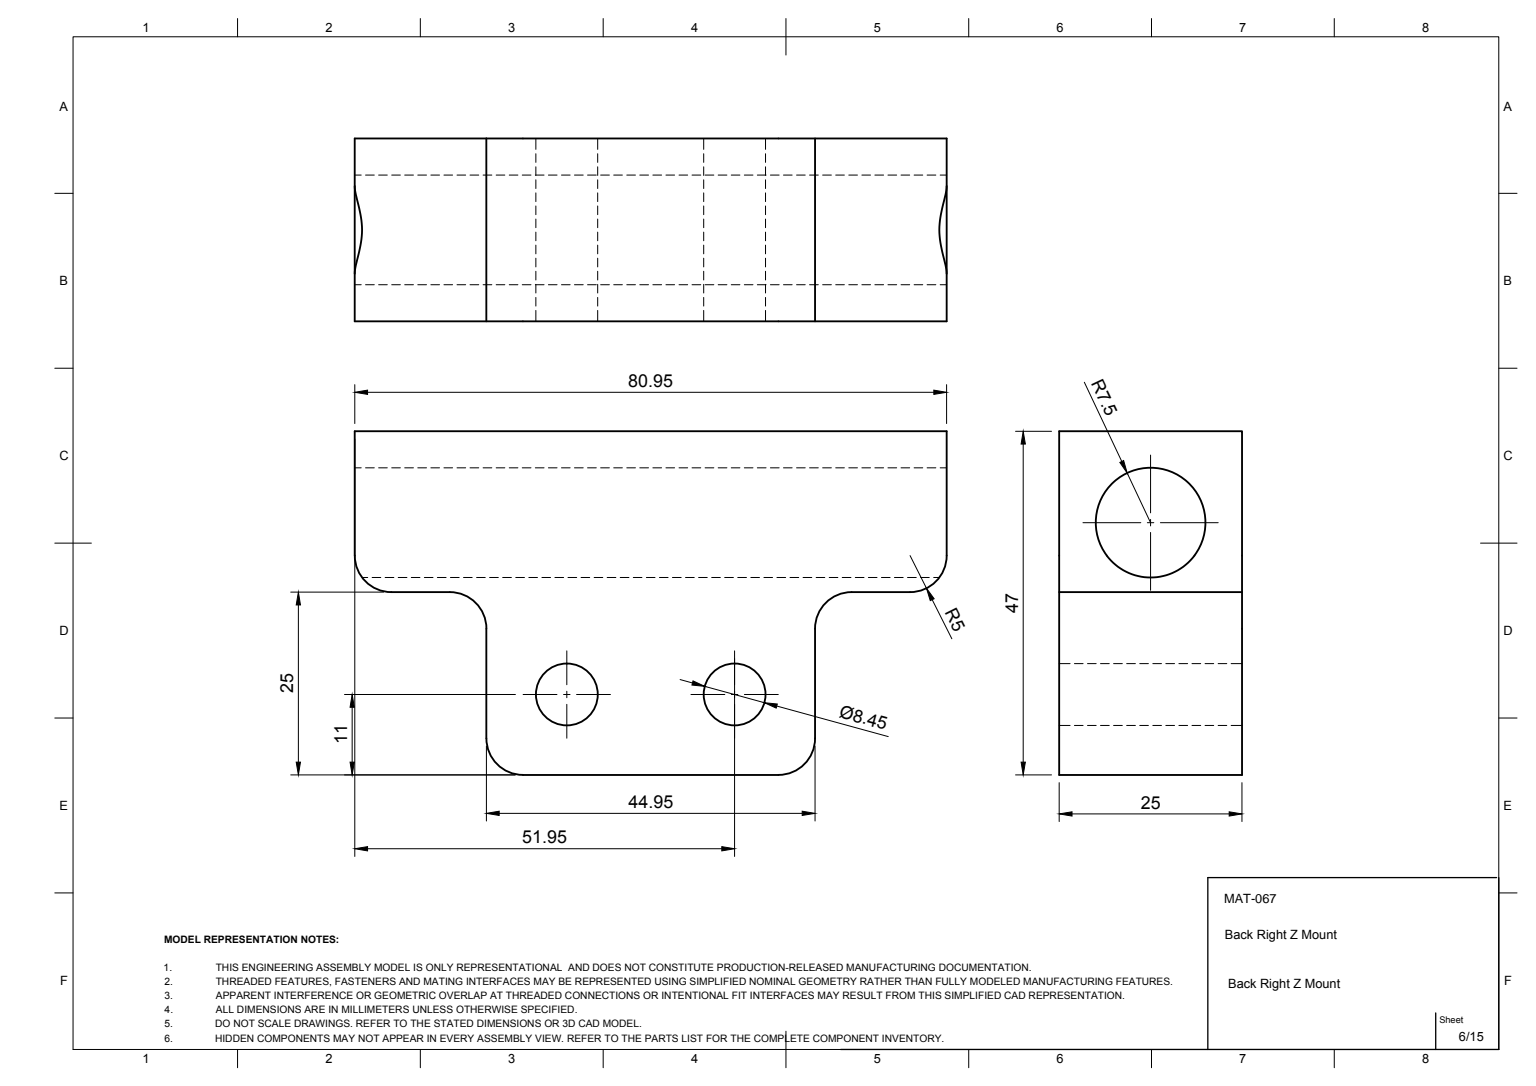
ISO-10303-21;
HEADER;
/* Generated by software containing ST-Developer
 * from STEP Tools, Inc. (www.steptools.com) 
 */

FILE_DESCRIPTION(
/* description */ ('CAx-IF Rec.Pracs.---Representation and Presentation of Product Manufa
cturing Information (PMI)---4.0---2014-10-13'),
/* implementation_level */ '2;1');

FILE_NAME(
/* name */ 'Back Right Z Mount.step',
/* time_stamp */ '2026-10-24T16:02:03-07:00',
/* author */ (''),
/* organization */ (''),
/* preprocessor_version */ 'ST-DEVELOPER v20.2',
/* originating_system */ 'Autodesk Translation Framework v15.17.0.0',
/* authorisation */ '');

FILE_SCHEMA (('AP242_MANAGED_MODEL_BASED_3D_ENGINEERING_MIM_LF { 1 0 10303 442 2 1 4 }'));
ENDSEC;

DATA;
#10=MECHANICAL_DESIGN_GEOMETRIC_PRESENTATION_REPRESENTATION('',(#352),#6348);
#330=SHAPE_REPRESENTATION_RELATIONSHIP('SRR','None',#6480,#341);
#341=ADVANCED_BREP_SHAPE_REPRESENTATION('',(#363),#6328);
#352=STYLED_ITEM('',(#6601),#363);
#363=MANIFOLD_SOLID_BREP('Body1',#3391);
#377=B_SPLINE_CURVE_WITH_KNOTS('',3,(#5673,#5674,#5675,#5676,#5677,#5678,
#5679,#5680,#5681,#5682,#5683,#5684,#5685,#5686,#5687,#5688,#5689,#5690),
 .UNSPECIFIED.,.F.,.F.,(4,2,2,2,2,2,2,2,4),(-2.14352388719531,-2.06484634554612,
-1.76300355616504,-1.61208216147449,-1.46116076678395,-1.31023937209341,
-1.15931797740286,-0.857475188021775,-0.778797646372586),.UNSPECIFIED.);
#378=B_SPLINE_CURVE_WITH_KNOTS('',3,(#5692,#5693,#5694,#5695,#5696,#5697,
#5698,#5699,#5700,#5701,#5702,#5703,#5704,#5705,#5706,#5707,#5708,#5709),
 .UNSPECIFIED.,.F.,.F.,(4,2,2,2,2,2,2,2,4),(-5.06584542076321,-4.98716787911402,
-4.68532508973293,-4.53440369504239,-4.38348230035184,-4.2325609056613,
-4.08163951097076,-3.77979672158967,-3.70111917994048),.UNSPECIFIED.);
#412=CYLINDRICAL_SURFACE('',#3668,0.004225);
#413=CYLINDRICAL_SURFACE('',#3669,0.004225);
#414=CYLINDRICAL_SURFACE('',#3671,0.0075);
#415=CYLINDRICAL_SURFACE('',#3676,0.005);
#416=CYLINDRICAL_SURFACE('',#3677,0.005);
#417=CYLINDRICAL_SURFACE('',#3678,0.005);
#418=CYLINDRICAL_SURFACE('',#3679,0.005);
#419=CYLINDRICAL_SURFACE('',#3680,0.005);
#420=CYLINDRICAL_SURFACE('',#3681,0.005);
#476=FACE_BOUND('',#938,.T.);
#477=FACE_BOUND('',#939,.T.);
#478=FACE_BOUND('',#941,.T.);
#479=FACE_BOUND('',#942,.T.);
#566=CIRCLE('',#3645,0.0075);
#567=CIRCLE('',#3646,0.0075);
#568=CIRCLE('',#3648,0.0075);
#569=CIRCLE('',#3649,0.0075);
#570=CIRCLE('',#3651,0.005);
#571=CIRCLE('',#3652,0.005);
#572=CIRCLE('',#3653,0.005);
#573=CIRCLE('',#3654,0.005);
#574=CIRCLE('',#3655,0.005);
#575=CIRCLE('',#3656,0.005);
#576=CIRCLE('',#3657,0.004225);
#577=CIRCLE('',#3658,0.004225);
#578=CIRCLE('',#3660,0.005);
#579=CIRCLE('',#3661,0.005);
#580=CIRCLE('',#3662,0.005);
#581=CIRCLE('',#3663,0.005);
#582=CIRCLE('',#3664,0.005);
#583=CIRCLE('',#3665,0.005);
#584=CIRCLE('',#3666,0.004225);
#585=CIRCLE('',#3667,0.004225);
#751=FACE_OUTER_BOUND('',#934,.T.);
#752=FACE_OUTER_BOUND('',#935,.T.);
#753=FACE_OUTER_BOUND('',#936,.T.);
#754=FACE_OUTER_BOUND('',#937,.T.);
#755=FACE_OUTER_BOUND('',#940,.T.);
#756=FACE_OUTER_BOUND('',#943,.T.);
#757=FACE_OUTER_BOUND('',#944,.T.);
#758=FACE_OUTER_BOUND('',#945,.T.);
#759=FACE_OUTER_BOUND('',#946,.T.);
#760=FACE_OUTER_BOUND('',#947,.T.);
#761=FACE_OUTER_BOUND('',#948,.T.);
#762=FACE_OUTER_BOUND('',#949,.T.);
#763=FACE_OUTER_BOUND('',#950,.T.);
#764=FACE_OUTER_BOUND('',#951,.T.);
#765=FACE_OUTER_BOUND('',#952,.T.);
#766=FACE_OUTER_BOUND('',#953,.T.);
#767=FACE_OUTER_BOUND('',#954,.T.);
#768=FACE_OUTER_BOUND('',#955,.T.);
#769=FACE_OUTER_BOUND('',#956,.T.);
#934=EDGE_LOOP('',(#2609,#2610,#2611,#2612));
#935=EDGE_LOOP('',(#2613,#2614,#2615,#2616,#2617,#2618,#2619));
#936=EDGE_LOOP('',(#2620,#2621,#2622,#2623,#2624,#2625,#2626));
#937=EDGE_LOOP('',(#2627,#2628,#2629,#2630,#2631,#2632,#2633,#2634,#2635,
#2636,#2637,#2638,#2639,#2640));
#938=EDGE_LOOP('',(#2641));
#939=EDGE_LOOP('',(#2642));
#940=EDGE_LOOP('',(#2643,#2644,#2645,#2646,#2647,#2648,#2649,#2650,#2651,
#2652,#2653,#2654,#2655,#2656));
#941=EDGE_LOOP('',(#2657));
#942=EDGE_LOOP('',(#2658));
#943=EDGE_LOOP('',(#2659,#2660,#2661,#2662));
#944=EDGE_LOOP('',(#2663,#2664,#2665,#2666));
#945=EDGE_LOOP('',(#2667,#2668,#2669,#2670));
#946=EDGE_LOOP('',(#2671,#2672,#2673,#2674,#2675,#2676,#2677,#2678));
#947=EDGE_LOOP('',(#2679,#2680,#2681,#2682));
#948=EDGE_LOOP('',(#2683,#2684,#2685,#2686));
#949=EDGE_LOOP('',(#2687,#2688,#2689,#2690));
#950=EDGE_LOOP('',(#2691,#2692,#2693,#2694));
#951=EDGE_LOOP('',(#2695,#2696,#2697,#2698));
#952=EDGE_LOOP('',(#2699,#2700,#2701,#2702,#2703,#2704));
#953=EDGE_LOOP('',(#2705,#2706,#2707,#2708));
#954=EDGE_LOOP('',(#2709,#2710,#2711,#2712,#2713,#2714));
#955=EDGE_LOOP('',(#2715,#2716,#2717,#2718));
#956=EDGE_LOOP('',(#2719,#2720,#2721,#2722));
#1183=LINE('',#5583,#1416);
#1184=LINE('',#5585,#1417);
#1185=LINE('',#5587,#1418);
#1186=LINE('',#5588,#1419);
#1187=LINE('',#5592,#1420);
#1188=LINE('',#5594,#1421);
#1189=LINE('',#5600,#1422);
#1190=LINE('',#5602,#1423);
#1191=LINE('',#5603,#1424);
#1192=LINE('',#5607,#1425);
#1193=LINE('',#5609,#1426);
#1194=LINE('',#5615,#1427);
#1195=LINE('',#5617,#1428);
#1196=LINE('',#5618,#1429);
#1197=LINE('',#5623,#1430);
#1198=LINE('',#5627,#1431);
#1199=LINE('',#5629,#1432);
#1200=LINE('',#5633,#1433);
#1201=LINE('',#5637,#1434);
#1202=LINE('',#5646,#1435);
#1203=LINE('',#5651,#1436);
#1204=LINE('',#5655,#1437);
#1205=LINE('',#5657,#1438);
#1206=LINE('',#5661,#1439);
#1207=LINE('',#5668,#1440);
#1208=LINE('',#5670,#1441);
#1209=LINE('',#5691,#1442);
#1210=LINE('',#5711,#1443);
#1211=LINE('',#5712,#1444);
#1212=LINE('',#5714,#1445);
#1213=LINE('',#5715,#1446);
#1214=LINE('',#5717,#1447);
#1215=LINE('',#5718,#1448);
#1216=LINE('',#5720,#1449);
#1217=LINE('',#5721,#1450);
#1416=VECTOR('',#4331,1.);
#1417=VECTOR('',#4332,1.);
#1418=VECTOR('',#4333,1.);
#1419=VECTOR('',#4334,1.);
#1420=VECTOR('',#4337,1.);
#1421=VECTOR('',#4338,1.);
#1422=VECTOR('',#4343,1.);
#1423=VECTOR('',#4344,1.);
#1424=VECTOR('',#4345,1.);
#1425=VECTOR('',#4348,1.);
#1426=VECTOR('',#4349,1.);
#1427=VECTOR('',#4354,1.);
#1428=VECTOR('',#4355,1.);
#1429=VECTOR('',#4356,1.);
#1430=VECTOR('',#4361,1.);
#1431=VECTOR('',#4364,1.);
#1432=VECTOR('',#4367,1.);
#1433=VECTOR('',#4370,1.);
#1434=VECTOR('',#4373,1.);
#1435=VECTOR('',#4382,1.);
#1436=VECTOR('',#4387,1.);
#1437=VECTOR('',#4390,1.);
#1438=VECTOR('',#4393,1.);
#1439=VECTOR('',#4396,1.);
#1440=VECTOR('',#4405,0.004225);
#1441=VECTOR('',#4408,0.004225);
#1442=VECTOR('',#4413,0.0075);
#1443=VECTOR('',#4416,1.);
#1444=VECTOR('',#4417,1.);
#1445=VECTOR('',#4420,1.);
#1446=VECTOR('',#4421,1.);
#1447=VECTOR('',#4424,1.);
#1448=VECTOR('',#4425,1.);
#1449=VECTOR('',#4428,1.);
#1450=VECTOR('',#4429,1.);
#1658=VERTEX_POINT('',#5581);
#1659=VERTEX_POINT('',#5582);
#1660=VERTEX_POINT('',#5584);
#1661=VERTEX_POINT('',#5586);
#1662=VERTEX_POINT('',#5590);
#1663=VERTEX_POINT('',#5591);
#1664=VERTEX_POINT('',#5593);
#1665=VERTEX_POINT('',#5595);
#1666=VERTEX_POINT('',#5597);
#1667=VERTEX_POINT('',#5599);
#1668=VERTEX_POINT('',#5601);
#1669=VERTEX_POINT('',#5605);
#1670=VERTEX_POINT('',#5606);
#1671=VERTEX_POINT('',#5608);
#1672=VERTEX_POINT('',#5610);
#1673=VERTEX_POINT('',#5612);
#1674=VERTEX_POINT('',#5614);
#1675=VERTEX_POINT('',#5616);
#1676=VERTEX_POINT('',#5620);
#1677=VERTEX_POINT('',#5622);
#1678=VERTEX_POINT('',#5624);
#1679=VERTEX_POINT('',#5626);
#1680=VERTEX_POINT('',#5630);
#1681=VERTEX_POINT('',#5632);
#1682=VERTEX_POINT('',#5634);
#1683=VERTEX_POINT('',#5636);
#1684=VERTEX_POINT('',#5639);
#1685=VERTEX_POINT('',#5641);
#1686=VERTEX_POINT('',#5644);
#1687=VERTEX_POINT('',#5645);
#1688=VERTEX_POINT('',#5648);
#1689=VERTEX_POINT('',#5650);
#1690=VERTEX_POINT('',#5652);
#1691=VERTEX_POINT('',#5654);
#1692=VERTEX_POINT('',#5658);
#1693=VERTEX_POINT('',#5660);
#1694=VERTEX_POINT('',#5663);
#1695=VERTEX_POINT('',#5665);
#2003=EDGE_CURVE('',#1658,#1659,#1183,.T.);
#2004=EDGE_CURVE('',#1659,#1660,#1184,.T.);
#2005=EDGE_CURVE('',#1661,#1660,#1185,.T.);
#2006=EDGE_CURVE('',#1661,#1658,#1186,.F.);
#2007=EDGE_CURVE('',#1662,#1663,#1187,.T.);
#2008=EDGE_CURVE('',#1662,#1664,#1188,.F.);
#2009=EDGE_CURVE('',#1664,#1665,#566,.T.);
#2010=EDGE_CURVE('',#1665,#1666,#567,.T.);
#2011=EDGE_CURVE('',#1666,#1667,#1189,.F.);
#2012=EDGE_CURVE('',#1667,#1668,#1190,.T.);
#2013=EDGE_CURVE('',#1663,#1668,#1191,.T.);
#2014=EDGE_CURVE('',#1669,#1670,#1192,.T.);
#2015=EDGE_CURVE('',#1669,#1671,#1193,.T.);
#2016=EDGE_CURVE('',#1672,#1671,#568,.T.);
#2017=EDGE_CURVE('',#1673,#1672,#569,.T.);
#2018=EDGE_CURVE('',#1673,#1674,#1194,.T.);
#2019=EDGE_CURVE('',#1674,#1675,#1195,.T.);
#2020=EDGE_CURVE('',#1675,#1670,#1196,.T.);
#2021=EDGE_CURVE('',#1660,#1676,#570,.T.);
#2022=EDGE_CURVE('',#1676,#1677,#1197,.T.);
#2023=EDGE_CURVE('',#1677,#1678,#571,.F.);
#2024=EDGE_CURVE('',#1679,#1678,#1198,.T.);
#2025=EDGE_CURVE('',#1679,#1662,#572,.T.);
#2026=EDGE_CURVE('',#1675,#1663,#1199,.T.);
#2027=EDGE_CURVE('',#1674,#1680,#573,.T.);
#2028=EDGE_CURVE('',#1680,#1681,#1200,.T.);
#2029=EDGE_CURVE('',#1681,#1682,#574,.F.);
#2030=EDGE_CURVE('',#1683,#1682,#1201,.T.);
#2031=EDGE_CURVE('',#1683,#1661,#575,.T.);
#2032=EDGE_CURVE('',#1684,#1684,#576,.T.);
#2033=EDGE_CURVE('',#1685,#1685,#577,.T.);
#2034=EDGE_CURVE('',#1686,#1687,#1202,.T.);
#2035=EDGE_CURVE('',#1686,#1659,#578,.F.);
#2036=EDGE_CURVE('',#1658,#1688,#579,.F.);
#2037=EDGE_CURVE('',#1688,#1689,#1203,.T.);
#2038=EDGE_CURVE('',#1689,#1690,#580,.T.);
#2039=EDGE_CURVE('',#1691,#1690,#1204,.T.);
#2040=EDGE_CURVE('',#1691,#1669,#581,.F.);
#2041=EDGE_CURVE('',#1670,#1668,#1205,.T.);
#2042=EDGE_CURVE('',#1667,#1692,#582,.F.);
#2043=EDGE_CURVE('',#1692,#1693,#1206,.T.);
#2044=EDGE_CURVE('',#1693,#1687,#583,.T.);
#2045=EDGE_CURVE('',#1694,#1694,#584,.T.);
#2046=EDGE_CURVE('',#1695,#1695,#585,.T.);
#2047=EDGE_CURVE('',#1684,#1694,#1207,.T.);
#2048=EDGE_CURVE('',#1685,#1695,#1208,.T.);
#2049=EDGE_CURVE('',#1664,#1666,#377,.T.);
#2050=EDGE_CURVE('',#1665,#1672,#1209,.T.);
#2051=EDGE_CURVE('',#1671,#1673,#378,.T.);
#2052=EDGE_CURVE('',#1676,#1686,#1210,.F.);
#2053=EDGE_CURVE('',#1687,#1677,#1211,.T.);
#2054=EDGE_CURVE('',#1692,#1679,#1212,.T.);
#2055=EDGE_CURVE('',#1678,#1693,#1213,.F.);
#2056=EDGE_CURVE('',#1682,#1689,#1214,.F.);
#2057=EDGE_CURVE('',#1688,#1683,#1215,.T.);
#2058=EDGE_CURVE('',#1680,#1691,#1216,.F.);
#2059=EDGE_CURVE('',#1690,#1681,#1217,.T.);
#2609=ORIENTED_EDGE('',*,*,#2003,.T.);
#2610=ORIENTED_EDGE('',*,*,#2004,.T.);
#2611=ORIENTED_EDGE('',*,*,#2005,.F.);
#2612=ORIENTED_EDGE('',*,*,#2006,.T.);
#2613=ORIENTED_EDGE('',*,*,#2007,.F.);
#2614=ORIENTED_EDGE('',*,*,#2008,.T.);
#2615=ORIENTED_EDGE('',*,*,#2009,.T.);
#2616=ORIENTED_EDGE('',*,*,#2010,.T.);
#2617=ORIENTED_EDGE('',*,*,#2011,.T.);
#2618=ORIENTED_EDGE('',*,*,#2012,.T.);
#2619=ORIENTED_EDGE('',*,*,#2013,.F.);
#2620=ORIENTED_EDGE('',*,*,#2014,.F.);
#2621=ORIENTED_EDGE('',*,*,#2015,.T.);
#2622=ORIENTED_EDGE('',*,*,#2016,.F.);
#2623=ORIENTED_EDGE('',*,*,#2017,.F.);
#2624=ORIENTED_EDGE('',*,*,#2018,.T.);
#2625=ORIENTED_EDGE('',*,*,#2019,.T.);
#2626=ORIENTED_EDGE('',*,*,#2020,.T.);
#2627=ORIENTED_EDGE('',*,*,#2005,.T.);
#2628=ORIENTED_EDGE('',*,*,#2021,.T.);
#2629=ORIENTED_EDGE('',*,*,#2022,.T.);
#2630=ORIENTED_EDGE('',*,*,#2023,.T.);
#2631=ORIENTED_EDGE('',*,*,#2024,.F.);
#2632=ORIENTED_EDGE('',*,*,#2025,.T.);
#2633=ORIENTED_EDGE('',*,*,#2007,.T.);
#2634=ORIENTED_EDGE('',*,*,#2026,.F.);
#2635=ORIENTED_EDGE('',*,*,#2019,.F.);
#2636=ORIENTED_EDGE('',*,*,#2027,.T.);
#2637=ORIENTED_EDGE('',*,*,#2028,.T.);
#2638=ORIENTED_EDGE('',*,*,#2029,.T.);
#2639=ORIENTED_EDGE('',*,*,#2030,.F.);
#2640=ORIENTED_EDGE('',*,*,#2031,.T.);
#2641=ORIENTED_EDGE('',*,*,#2032,.F.);
#2642=ORIENTED_EDGE('',*,*,#2033,.F.);
#2643=ORIENTED_EDGE('',*,*,#2034,.F.);
#2644=ORIENTED_EDGE('',*,*,#2035,.T.);
#2645=ORIENTED_EDGE('',*,*,#2003,.F.);
#2646=ORIENTED_EDGE('',*,*,#2036,.T.);
#2647=ORIENTED_EDGE('',*,*,#2037,.T.);
#2648=ORIENTED_EDGE('',*,*,#2038,.T.);
#2649=ORIENTED_EDGE('',*,*,#2039,.F.);
#2650=ORIENTED_EDGE('',*,*,#2040,.T.);
#2651=ORIENTED_EDGE('',*,*,#2014,.T.);
#2652=ORIENTED_EDGE('',*,*,#2041,.T.);
#2653=ORIENTED_EDGE('',*,*,#2012,.F.);
#2654=ORIENTED_EDGE('',*,*,#2042,.T.);
#2655=ORIENTED_EDGE('',*,*,#2043,.T.);
#2656=ORIENTED_EDGE('',*,*,#2044,.T.);
#2657=ORIENTED_EDGE('',*,*,#2045,.T.);
#2658=ORIENTED_EDGE('',*,*,#2046,.T.);
#2659=ORIENTED_EDGE('',*,*,#2032,.T.);
#2660=ORIENTED_EDGE('',*,*,#2047,.T.);
#2661=ORIENTED_EDGE('',*,*,#2045,.F.);
#2662=ORIENTED_EDGE('',*,*,#2047,.F.);
#2663=ORIENTED_EDGE('',*,*,#2033,.T.);
#2664=ORIENTED_EDGE('',*,*,#2048,.T.);
#2665=ORIENTED_EDGE('',*,*,#2046,.F.);
#2666=ORIENTED_EDGE('',*,*,#2048,.F.);
#2667=ORIENTED_EDGE('',*,*,#2041,.F.);
#2668=ORIENTED_EDGE('',*,*,#2020,.F.);
#2669=ORIENTED_EDGE('',*,*,#2026,.T.);
#2670=ORIENTED_EDGE('',*,*,#2013,.T.);
#2671=ORIENTED_EDGE('',*,*,#2009,.F.);
#2672=ORIENTED_EDGE('',*,*,#2049,.T.);
#2673=ORIENTED_EDGE('',*,*,#2010,.F.);
#2674=ORIENTED_EDGE('',*,*,#2050,.T.);
#2675=ORIENTED_EDGE('',*,*,#2016,.T.);
#2676=ORIENTED_EDGE('',*,*,#2051,.T.);
#2677=ORIENTED_EDGE('',*,*,#2017,.T.);
#2678=ORIENTED_EDGE('',*,*,#2050,.F.);
#2679=ORIENTED_EDGE('',*,*,#2022,.F.);
#2680=ORIENTED_EDGE('',*,*,#2052,.T.);
#2681=ORIENTED_EDGE('',*,*,#2034,.T.);
#2682=ORIENTED_EDGE('',*,*,#2053,.T.);
#2683=ORIENTED_EDGE('',*,*,#2043,.F.);
#2684=ORIENTED_EDGE('',*,*,#2054,.T.);
#2685=ORIENTED_EDGE('',*,*,#2024,.T.);
#2686=ORIENTED_EDGE('',*,*,#2055,.T.);
#2687=ORIENTED_EDGE('',*,*,#2030,.T.);
#2688=ORIENTED_EDGE('',*,*,#2056,.T.);
#2689=ORIENTED_EDGE('',*,*,#2037,.F.);
#2690=ORIENTED_EDGE('',*,*,#2057,.T.);
#2691=ORIENTED_EDGE('',*,*,#2028,.F.);
#2692=ORIENTED_EDGE('',*,*,#2058,.T.);
#2693=ORIENTED_EDGE('',*,*,#2039,.T.);
#2694=ORIENTED_EDGE('',*,*,#2059,.T.);
#2695=ORIENTED_EDGE('',*,*,#2035,.F.);
#2696=ORIENTED_EDGE('',*,*,#2052,.F.);
#2697=ORIENTED_EDGE('',*,*,#2021,.F.);
#2698=ORIENTED_EDGE('',*,*,#2004,.F.);
#2699=ORIENTED_EDGE('',*,*,#2049,.F.);
#2700=ORIENTED_EDGE('',*,*,#2008,.F.);
#2701=ORIENTED_EDGE('',*,*,#2025,.F.);
#2702=ORIENTED_EDGE('',*,*,#2054,.F.);
#2703=ORIENTED_EDGE('',*,*,#2042,.F.);
#2704=ORIENTED_EDGE('',*,*,#2011,.F.);
#2705=ORIENTED_EDGE('',*,*,#2044,.F.);
#2706=ORIENTED_EDGE('',*,*,#2055,.F.);
#2707=ORIENTED_EDGE('',*,*,#2023,.F.);
#2708=ORIENTED_EDGE('',*,*,#2053,.F.);
#2709=ORIENTED_EDGE('',*,*,#2040,.F.);
#2710=ORIENTED_EDGE('',*,*,#2058,.F.);
#2711=ORIENTED_EDGE('',*,*,#2027,.F.);
#2712=ORIENTED_EDGE('',*,*,#2018,.F.);
#2713=ORIENTED_EDGE('',*,*,#2051,.F.);
#2714=ORIENTED_EDGE('',*,*,#2015,.F.);
#2715=ORIENTED_EDGE('',*,*,#2038,.F.);
#2716=ORIENTED_EDGE('',*,*,#2056,.F.);
#2717=ORIENTED_EDGE('',*,*,#2029,.F.);
#2718=ORIENTED_EDGE('',*,*,#2059,.F.);
#2719=ORIENTED_EDGE('',*,*,#2036,.F.);
#2720=ORIENTED_EDGE('',*,*,#2006,.F.);
#2721=ORIENTED_EDGE('',*,*,#2031,.F.);
#2722=ORIENTED_EDGE('',*,*,#2057,.F.);
#3167=PLANE('',#3643);
#3168=PLANE('',#3644);
#3169=PLANE('',#3647);
#3170=PLANE('',#3650);
#3171=PLANE('',#3659);
#3172=PLANE('',#3670);
#3173=PLANE('',#3672);
#3174=PLANE('',#3673);
#3175=PLANE('',#3674);
#3176=PLANE('',#3675);
#3274=ADVANCED_FACE('',(#751),#3167,.F.);
#3275=ADVANCED_FACE('',(#752),#3168,.F.);
#3276=ADVANCED_FACE('',(#753),#3169,.T.);
#3277=ADVANCED_FACE('',(#754,#476,#477),#3170,.T.);
#3278=ADVANCED_FACE('',(#755,#478,#479),#3171,.F.);
#3279=ADVANCED_FACE('',(#756),#412,.F.);
#3280=ADVANCED_FACE('',(#757),#413,.F.);
#3281=ADVANCED_FACE('',(#758),#3172,.T.);
#3282=ADVANCED_FACE('',(#759),#414,.F.);
#3283=ADVANCED_FACE('',(#760),#3173,.T.);
#3284=ADVANCED_FACE('',(#761),#3174,.F.);
#3285=ADVANCED_FACE('',(#762),#3175,.F.);
#3286=ADVANCED_FACE('',(#763),#3176,.T.);
#3287=ADVANCED_FACE('',(#764),#415,.T.);
#3288=ADVANCED_FACE('',(#765),#416,.T.);
#3289=ADVANCED_FACE('',(#766),#417,.F.);
#3290=ADVANCED_FACE('',(#767),#418,.T.);
#3291=ADVANCED_FACE('',(#768),#419,.F.);
#3292=ADVANCED_FACE('',(#769),#420,.T.);
#3391=CLOSED_SHELL('',(#3274,#3275,#3276,#3277,#3278,#3279,#3280,#3281,
#3282,#3283,#3284,#3285,#3286,#3287,#3288,#3289,#3290,#3291,#3292));
#3642=AXIS2_PLACEMENT_3D('',#5579,#4327,#4328);
#3643=AXIS2_PLACEMENT_3D('',#5580,#4329,#4330);
#3644=AXIS2_PLACEMENT_3D('',#5589,#4335,#4336);
#3645=AXIS2_PLACEMENT_3D('',#5596,#4339,#4340);
#3646=AXIS2_PLACEMENT_3D('',#5598,#4341,#4342);
#3647=AXIS2_PLACEMENT_3D('',#5604,#4346,#4347);
#3648=AXIS2_PLACEMENT_3D('',#5611,#4350,#4351);
#3649=AXIS2_PLACEMENT_3D('',#5613,#4352,#4353);
#3650=AXIS2_PLACEMENT_3D('',#5619,#4357,#4358);
#3651=AXIS2_PLACEMENT_3D('',#5621,#4359,#4360);
#3652=AXIS2_PLACEMENT_3D('',#5625,#4362,#4363);
#3653=AXIS2_PLACEMENT_3D('',#5628,#4365,#4366);
#3654=AXIS2_PLACEMENT_3D('',#5631,#4368,#4369);
#3655=AXIS2_PLACEMENT_3D('',#5635,#4371,#4372);
#3656=AXIS2_PLACEMENT_3D('',#5638,#4374,#4375);
#3657=AXIS2_PLACEMENT_3D('',#5640,#4376,#4377);
#3658=AXIS2_PLACEMENT_3D('',#5642,#4378,#4379);
#3659=AXIS2_PLACEMENT_3D('',#5643,#4380,#4381);
#3660=AXIS2_PLACEMENT_3D('',#5647,#4383,#4384);
#3661=AXIS2_PLACEMENT_3D('',#5649,#4385,#4386);
#3662=AXIS2_PLACEMENT_3D('',#5653,#4388,#4389);
#3663=AXIS2_PLACEMENT_3D('',#5656,#4391,#4392);
#3664=AXIS2_PLACEMENT_3D('',#5659,#4394,#4395);
#3665=AXIS2_PLACEMENT_3D('',#5662,#4397,#4398);
#3666=AXIS2_PLACEMENT_3D('',#5664,#4399,#4400);
#3667=AXIS2_PLACEMENT_3D('',#5666,#4401,#4402);
#3668=AXIS2_PLACEMENT_3D('',#5667,#4403,#4404);
#3669=AXIS2_PLACEMENT_3D('',#5669,#4406,#4407);
#3670=AXIS2_PLACEMENT_3D('',#5671,#4409,#4410);
#3671=AXIS2_PLACEMENT_3D('',#5672,#4411,#4412);
#3672=AXIS2_PLACEMENT_3D('',#5710,#4414,#4415);
#3673=AXIS2_PLACEMENT_3D('',#5713,#4418,#4419);
#3674=AXIS2_PLACEMENT_3D('',#5716,#4422,#4423);
#3675=AXIS2_PLACEMENT_3D('',#5719,#4426,#4427);
#3676=AXIS2_PLACEMENT_3D('',#5722,#4430,#4431);
#3677=AXIS2_PLACEMENT_3D('',#5723,#4432,#4433);
#3678=AXIS2_PLACEMENT_3D('',#5724,#4434,#4435);
#3679=AXIS2_PLACEMENT_3D('',#5725,#4436,#4437);
#3680=AXIS2_PLACEMENT_3D('',#5726,#4438,#4439);
#3681=AXIS2_PLACEMENT_3D('',#5727,#4440,#4441);
#4327=DIRECTION('axis',(0.,0.,1.));
#4328=DIRECTION('refdir',(1.,0.,0.));
#4329=DIRECTION('center_axis',(-1.,0.,0.));
#4330=DIRECTION('ref_axis',(0.,0.,-1.));
#4331=DIRECTION('',(0.,8.57182693503055E-17,-1.));
#4332=DIRECTION('',(0.,1.,8.57182693503055E-17));
#4333=DIRECTION('',(0.,8.57182693503055E-17,-1.));
#4334=DIRECTION('',(0.,1.,8.57182693503055E-17));
#4335=DIRECTION('center_axis',(0.,-8.57182693503055E-17,1.));
#4336=DIRECTION('ref_axis',(0.,1.,8.57182693503055E-17));
#4337=DIRECTION('',(-1.,0.,0.));
#4338=DIRECTION('',(0.,1.,8.57182693503055E-17));
#4339=DIRECTION('center_axis',(0.,-8.57182693503055E-17,1.));
#4340=DIRECTION('ref_axis',(0.,1.,8.57182693503055E-17));
#4341=DIRECTION('center_axis',(0.,-8.57182693503055E-17,1.));
#4342=DIRECTION('ref_axis',(0.,1.,8.57182693503055E-17));
#4343=DIRECTION('',(0.,1.,8.57182693503055E-17));
#4344=DIRECTION('',(-1.,0.,0.));
#4345=DIRECTION('',(0.,-1.,-8.57182693503055E-17));
#4346=DIRECTION('center_axis',(0.,-8.57182693503055E-17,1.));
#4347=DIRECTION('ref_axis',(0.,1.,8.57182693503055E-17));
#4348=DIRECTION('',(-1.,0.,0.));
#4349=DIRECTION('',(0.,1.,8.57182693503055E-17));
#4350=DIRECTION('center_axis',(0.,-8.57182693503055E-17,1.));
#4351=DIRECTION('ref_axis',(0.,1.,8.57182693503055E-17));
#4352=DIRECTION('center_axis',(0.,-8.57182693503055E-17,1.));
#4353=DIRECTION('ref_axis',(0.,1.,8.57182693503055E-17));
#4354=DIRECTION('',(0.,1.,8.57182693503055E-17));
#4355=DIRECTION('',(-1.,0.,0.));
#4356=DIRECTION('',(0.,-1.,-8.57182693503055E-17));
#4357=DIRECTION('center_axis',(0.,1.,8.57182693503055E-17));
#4358=DIRECTION('ref_axis',(-1.,0.,0.));
#4359=DIRECTION('center_axis',(0.,1.,8.57182693503055E-17));
#4360=DIRECTION('ref_axis',(0.,8.57182693503055E-17,-1.));
#4361=DIRECTION('',(-1.,0.,0.));
#4362=DIRECTION('center_axis',(0.,1.,8.57182693503055E-17));
#4363=DIRECTION('ref_axis',(0.,8.57182693503055E-17,-1.));
#4364=DIRECTION('',(0.,-8.57182693503055E-17,1.));
#4365=DIRECTION('center_axis',(0.,1.,8.57182693503055E-17));
#4366=DIRECTION('ref_axis',(0.,8.57182693503055E-17,-1.));
#4367=DIRECTION('',(0.,8.57182693503055E-17,-1.));
#4368=DIRECTION('center_axis',(0.,1.,8.57182693503055E-17));
#4369=DIRECTION('ref_axis',(0.,8.57182693503055E-17,-1.));
#4370=DIRECTION('',(0.,8.57182693503055E-17,-1.));
#4371=DIRECTION('center_axis',(0.,1.,8.57182693503055E-17));
#4372=DIRECTION('ref_axis',(0.,8.57182693503055E-17,-1.));
#4373=DIRECTION('',(-1.,0.,0.));
#4374=DIRECTION('center_axis',(0.,1.,8.57182693503055E-17));
#4375=DIRECTION('ref_axis',(0.,8.57182693503055E-17,-1.));
#4376=DIRECTION('center_axis',(0.,1.,8.57182693503055E-17));
#4377=DIRECTION('ref_axis',(0.,8.57182693503055E-17,-1.));
#4378=DIRECTION('center_axis',(0.,1.,8.57182693503055E-17));
#4379=DIRECTION('ref_axis',(0.,8.57182693503055E-17,-1.));
#4380=DIRECTION('center_axis',(0.,1.,8.57182693503055E-17));
#4381=DIRECTION('ref_axis',(-1.,0.,0.));
#4382=DIRECTION('',(-1.,0.,0.));
#4383=DIRECTION('center_axis',(0.,1.,8.57182693503055E-17));
#4384=DIRECTION('ref_axis',(0.,8.57182693503055E-17,-1.));
#4385=DIRECTION('center_axis',(0.,1.,8.57182693503055E-17));
#4386=DIRECTION('ref_axis',(0.,8.57182693503055E-17,-1.));
#4387=DIRECTION('',(-1.,0.,0.));
#4388=DIRECTION('center_axis',(0.,1.,8.57182693503055E-17));
#4389=DIRECTION('ref_axis',(0.,8.57182693503055E-17,-1.));
#4390=DIRECTION('',(0.,8.57182693503055E-17,-1.));
#4391=DIRECTION('center_axis',(0.,1.,8.57182693503055E-17));
#4392=DIRECTION('ref_axis',(0.,8.57182693503055E-17,-1.));
#4393=DIRECTION('',(0.,8.57182693503055E-17,-1.));
#4394=DIRECTION('center_axis',(0.,1.,8.57182693503055E-17));
#4395=DIRECTION('ref_axis',(0.,8.57182693503055E-17,-1.));
#4396=DIRECTION('',(0.,-8.57182693503055E-17,1.));
#4397=DIRECTION('center_axis',(0.,1.,8.57182693503055E-17));
#4398=DIRECTION('ref_axis',(0.,8.57182693503055E-17,-1.));
#4399=DIRECTION('center_axis',(0.,1.,8.57182693503055E-17));
#4400=DIRECTION('ref_axis',(0.,8.57182693503055E-17,-1.));
#4401=DIRECTION('center_axis',(0.,1.,8.57182693503055E-17));
#4402=DIRECTION('ref_axis',(0.,8.57182693503055E-17,-1.));
#4403=DIRECTION('center_axis',(0.,-1.,-8.57182693503055E-17));
#4404=DIRECTION('ref_axis',(0.,-8.57182693503055E-17,1.));
#4405=DIRECTION('',(0.,-1.,-8.57182693503055E-17));
#4406=DIRECTION('center_axis',(0.,-1.,-8.57182693503055E-17));
#4407=DIRECTION('ref_axis',(0.,-8.57182693503055E-17,1.));
#4408=DIRECTION('',(0.,-1.,-8.57182693503055E-17));
#4409=DIRECTION('center_axis',(-1.,0.,0.));
#4410=DIRECTION('ref_axis',(0.,0.,-1.));
#4411=DIRECTION('center_axis',(0.,-8.57182693503055E-17,1.));
#4412=DIRECTION('ref_axis',(0.,1.,8.57182693503055E-17));
#4413=DIRECTION('',(0.,-8.57182693503055E-17,1.));
#4414=DIRECTION('center_axis',(0.,8.57182693503055E-17,-1.));
#4415=DIRECTION('ref_axis',(0.,-1.,-8.57182693503055E-17));
#4416=DIRECTION('',(0.,1.,8.57182693503055E-17));
#4417=DIRECTION('',(0.,1.,8.57182693503055E-17));
#4418=DIRECTION('center_axis',(-1.,0.,0.));
#4419=DIRECTION('ref_axis',(0.,0.,-1.));
#4420=DIRECTION('',(0.,1.,8.57182693503055E-17));
#4421=DIRECTION('',(0.,1.,8.57182693503055E-17));
#4422=DIRECTION('center_axis',(0.,8.57182693503055E-17,-1.));
#4423=DIRECTION('ref_axis',(0.,-1.,-8.57182693503055E-17));
#4424=DIRECTION('',(0.,1.,8.57182693503055E-17));
#4425=DIRECTION('',(0.,1.,8.57182693503055E-17));
#4426=DIRECTION('center_axis',(1.,0.,0.));
#4427=DIRECTION('ref_axis',(0.,0.,1.));
#4428=DIRECTION('',(0.,1.,8.57182693503055E-17));
#4429=DIRECTION('',(0.,1.,8.57182693503055E-17));
#4430=DIRECTION('center_axis',(0.,-1.,-8.57182693503055E-17));
#4431=DIRECTION('ref_axis',(0.,-8.57182693503055E-17,1.));
#4432=DIRECTION('center_axis',(0.,1.,8.57182693503055E-17));
#4433=DIRECTION('ref_axis',(0.,8.57182693503055E-17,-1.));
#4434=DIRECTION('center_axis',(0.,1.,8.57182693503055E-17));
#4435=DIRECTION('ref_axis',(0.,8.57182693503055E-17,-1.));
#4436=DIRECTION('center_axis',(0.,1.,8.57182693503055E-17));
#4437=DIRECTION('ref_axis',(0.,8.57182693503055E-17,-1.));
#4438=DIRECTION('center_axis',(0.,1.,8.57182693503055E-17));
#4439=DIRECTION('ref_axis',(0.,8.57182693503055E-17,-1.));
#4440=DIRECTION('center_axis',(0.,1.,8.57182693503055E-17));
#4441=DIRECTION('ref_axis',(0.,8.57182693503055E-17,-1.));
#5579=CARTESIAN_POINT('',(0.,0.,0.));
#5580=CARTESIAN_POINT('Origin',(0.06855,0.1092,0.02565));
#5581=CARTESIAN_POINT('',(0.06855,0.0842,0.043125));
#5582=CARTESIAN_POINT('',(0.06855,0.0842,0.008175));
#5583=CARTESIAN_POINT('',(0.06855,0.0842,0.02565));
#5584=CARTESIAN_POINT('',(0.06855,0.1092,0.008175));
#5585=CARTESIAN_POINT('',(0.06855,0.1092,0.008175));
#5586=CARTESIAN_POINT('',(0.06855,0.1092,0.043125));
#5587=CARTESIAN_POINT('',(0.06855,0.1092,0.02565));
#5588=CARTESIAN_POINT('',(0.06855,0.1092,0.043125));
#5589=CARTESIAN_POINT('Origin',(0.05755,0.1092,-0.014825));
#5590=CARTESIAN_POINT('',(0.03855,0.1092,-0.014825));
#5591=CARTESIAN_POINT('',(0.02155,0.1092,-0.014825));
#5592=CARTESIAN_POINT('',(0.05755,0.1092,-0.014825));
#5593=CARTESIAN_POINT('',(0.03855,0.1027,-0.014825));
#5594=CARTESIAN_POINT('',(0.03855,0.1092,-0.014825));
#5595=CARTESIAN_POINT('',(0.03405,0.0892,-0.014825));
#5596=CARTESIAN_POINT('Origin',(0.03405,0.0967,-0.014825));
#5597=CARTESIAN_POINT('',(0.03855,0.0907,-0.014825));
#5598=CARTESIAN_POINT('Origin',(0.03405,0.0967,-0.014825));
#5599=CARTESIAN_POINT('',(0.03855,0.0842,-0.014825));
#5600=CARTESIAN_POINT('',(0.03855,0.1092,-0.014825));
#5601=CARTESIAN_POINT('',(0.02155,0.0842,-0.014825));
#5602=CARTESIAN_POINT('',(0.05755,0.0842,-0.014825));
#5603=CARTESIAN_POINT('',(0.02155,0.1092,-0.014825));
#5604=CARTESIAN_POINT('Origin',(0.05755,0.1092,0.066125));
#5605=CARTESIAN_POINT('',(0.03855,0.0842,0.066125));
#5606=CARTESIAN_POINT('',(0.02155,0.0842,0.066125));
#5607=CARTESIAN_POINT('',(0.05755,0.0842,0.066125));
#5608=CARTESIAN_POINT('',(0.03855,0.0907,0.066125));
#5609=CARTESIAN_POINT('',(0.03855,0.1092,0.066125));
#5610=CARTESIAN_POINT('',(0.03405,0.0892,0.066125));
#5611=CARTESIAN_POINT('Origin',(0.03405,0.0967,0.066125));
#5612=CARTESIAN_POINT('',(0.03855,0.1027,0.066125));
#5613=CARTESIAN_POINT('Origin',(0.03405,0.0967,0.066125));
#5614=CARTESIAN_POINT('',(0.03855,0.1092,0.066125));
#5615=CARTESIAN_POINT('',(0.03855,0.1092,0.066125));
#5616=CARTESIAN_POINT('',(0.02155,0.1092,0.066125));
#5617=CARTESIAN_POINT('',(0.05755,0.1092,0.066125));
#5618=CARTESIAN_POINT('',(0.02155,0.1092,0.066125));
#5619=CARTESIAN_POINT('Origin',(0.05755,0.1092,0.02565));
#5620=CARTESIAN_POINT('',(0.06355,0.1092,0.003175));
#5621=CARTESIAN_POINT('Origin',(0.06355,0.1092,0.008175));
#5622=CARTESIAN_POINT('',(0.04855,0.1092,0.003175));
#5623=CARTESIAN_POINT('',(0.05605,0.1092,0.003175));
#5624=CARTESIAN_POINT('',(0.04355,0.1092,-0.001825));
#5625=CARTESIAN_POINT('Origin',(0.04855,0.1092,-0.001825));
#5626=CARTESIAN_POINT('',(0.04355,0.1092,-0.009825));
#5627=CARTESIAN_POINT('',(0.04355,0.1092,-0.005825));
#5628=CARTESIAN_POINT('Origin',(0.03855,0.1092,-0.009825));
#5629=CARTESIAN_POINT('',(0.02155,0.1092,0.02565));
#5630=CARTESIAN_POINT('',(0.04355,0.1092,0.061125));
#5631=CARTESIAN_POINT('Origin',(0.03855,0.1092,0.061125));
#5632=CARTESIAN_POINT('',(0.04355,0.1092,0.053125));
#5633=CARTESIAN_POINT('',(0.04355,0.1092,0.057125));
#5634=CARTESIAN_POINT('',(0.04855,0.1092,0.048125));
#5635=CARTESIAN_POINT('Origin',(0.04855,0.1092,0.053125));
#5636=CARTESIAN_POINT('',(0.06355,0.1092,0.048125));
#5637=CARTESIAN_POINT('',(0.05605,0.1092,0.048125));
#5638=CARTESIAN_POINT('Origin',(0.06355,0.1092,0.043125));
#5639=CARTESIAN_POINT('',(0.05755,0.1092,0.0329));
#5640=CARTESIAN_POINT('Origin',(0.05755,0.1092,0.037125));
#5641=CARTESIAN_POINT('',(0.05755,0.1092,0.00995));
#5642=CARTESIAN_POINT('Origin',(0.05755,0.1092,0.014175));
#5643=CARTESIAN_POINT('Origin',(0.05755,0.0842,0.02565));
#5644=CARTESIAN_POINT('',(0.06355,0.0842,0.003175));
#5645=CARTESIAN_POINT('',(0.04855,0.0842,0.003175));
#5646=CARTESIAN_POINT('',(0.05605,0.0842,0.003175));
#5647=CARTESIAN_POINT('Origin',(0.06355,0.0842,0.008175));
#5648=CARTESIAN_POINT('',(0.06355,0.0842,0.048125));
#5649=CARTESIAN_POINT('Origin',(0.06355,0.0842,0.043125));
#5650=CARTESIAN_POINT('',(0.04855,0.0842,0.048125));
#5651=CARTESIAN_POINT('',(0.05605,0.0842,0.048125));
#5652=CARTESIAN_POINT('',(0.04355,0.0842,0.053125));
#5653=CARTESIAN_POINT('Origin',(0.04855,0.0842,0.053125));
#5654=CARTESIAN_POINT('',(0.04355,0.0842,0.061125));
#5655=CARTESIAN_POINT('',(0.04355,0.0842,0.057125));
#5656=CARTESIAN_POINT('Origin',(0.03855,0.0842,0.061125));
#5657=CARTESIAN_POINT('',(0.02155,0.0842,0.02565));
#5658=CARTESIAN_POINT('',(0.04355,0.0842,-0.009825));
#5659=CARTESIAN_POINT('Origin',(0.03855,0.0842,-0.009825));
#5660=CARTESIAN_POINT('',(0.04355,0.0842,-0.001825));
#5661=CARTESIAN_POINT('',(0.04355,0.0842,-0.005825));
#5662=CARTESIAN_POINT('Origin',(0.04855,0.0842,-0.001825));
#5663=CARTESIAN_POINT('',(0.05755,0.0842,0.0329));
#5664=CARTESIAN_POINT('Origin',(0.05755,0.0842,0.037125));
#5665=CARTESIAN_POINT('',(0.05755,0.0842,0.00995));
#5666=CARTESIAN_POINT('Origin',(0.05755,0.0842,0.014175));
#5667=CARTESIAN_POINT('Origin',(0.05755,0.1092,0.037125));
#5668=CARTESIAN_POINT('',(0.05755,0.1092,0.0329));
#5669=CARTESIAN_POINT('Origin',(0.05755,0.1092,0.014175));
#5670=CARTESIAN_POINT('',(0.05755,0.1092,0.00995));
#5671=CARTESIAN_POINT('Origin',(0.02155,0.1092,0.02565));
#5672=CARTESIAN_POINT('Origin',(0.03405,0.0967,-0.023875));
#5673=CARTESIAN_POINT('Ctrl Pts',(0.03855,0.1027,-0.014825));
#5674=CARTESIAN_POINT('Ctrl Pts',(0.0387729524989471,0.10253278562579,-0.014825));
#5675=CARTESIAN_POINT('Ctrl Pts',(0.0389827504953742,0.102355632371189,
-0.0148099450879691));
#5676=CARTESIAN_POINT('Ctrl Pts',(0.0399051826894431,0.101492776063005,
-0.0146940175331532));
#5677=CARTESIAN_POINT('Ctrl Pts',(0.0405168708018142,0.100636070492068,
-0.0144455865368071));
#5678=CARTESIAN_POINT('Ctrl Pts',(0.0411335425015076,0.0992177720348636,
-0.0141121811456859));
#5679=CARTESIAN_POINT('Ctrl Pts',(0.0412904479475092,0.0987224751365548,
-0.0140090151899698));
#5680=CARTESIAN_POINT('Ctrl Pts',(0.0414987473161672,0.0977152118956436,
-0.013864916792468));
#5681=CARTESIAN_POINT('Ctrl Pts',(0.04155,0.0972030713156352,-0.013825));
#5682=CARTESIAN_POINT('Ctrl Pts',(0.04155,0.0961969286843648,-0.013825));
#5683=CARTESIAN_POINT('Ctrl Pts',(0.0414987473161672,0.0956847881043564,
-0.013864916792468));
#5684=CARTESIAN_POINT('Ctrl Pts',(0.0412904479475093,0.0946775248634452,
-0.0140090151899698));
#5685=CARTESIAN_POINT('Ctrl Pts',(0.0411335425015076,0.0941822279651364,
-0.0141121811456859));
#5686=CARTESIAN_POINT('Ctrl Pts',(0.0405168708018142,0.0927639295079321,
-0.0144455865368071));
#5687=CARTESIAN_POINT('Ctrl Pts',(0.0399051826894431,0.0919072239369945,
-0.0146940175331532));
#5688=CARTESIAN_POINT('Ctrl Pts',(0.0389827504953742,0.0910443676288105,
-0.0148099450879691));
#5689=CARTESIAN_POINT('Ctrl Pts',(0.0387729524989471,0.0908672143742103,
-0.014825));
#5690=CARTESIAN_POINT('Ctrl Pts',(0.03855,0.0907,-0.014825));
#5691=CARTESIAN_POINT('',(0.03405,0.0892,-0.023875));
#5692=CARTESIAN_POINT('Ctrl Pts',(0.03855,0.0907,0.066125));
#5693=CARTESIAN_POINT('Ctrl Pts',(0.0387729524989471,0.0908672143742103,
0.066125));
#5694=CARTESIAN_POINT('Ctrl Pts',(0.0389827504953742,0.0910443676288105,
0.0661099450879691));
#5695=CARTESIAN_POINT('Ctrl Pts',(0.039905182689443,0.0919072239369945,
0.0659940175331532));
#5696=CARTESIAN_POINT('Ctrl Pts',(0.0405168708018142,0.0927639295079321,
0.0657455865368071));
#5697=CARTESIAN_POINT('Ctrl Pts',(0.0411335425015076,0.0941822279651364,
0.0654121811456859));
#5698=CARTESIAN_POINT('Ctrl Pts',(0.0412904479475093,0.0946775248634452,
0.0653090151899698));
#5699=CARTESIAN_POINT('Ctrl Pts',(0.0414987473161672,0.0956847881043564,
0.065164916792468));
#5700=CARTESIAN_POINT('Ctrl Pts',(0.04155,0.0961969286843649,0.065125));
#5701=CARTESIAN_POINT('Ctrl Pts',(0.04155,0.0972030713156351,0.065125));
#5702=CARTESIAN_POINT('Ctrl Pts',(0.0414987473161672,0.0977152118956436,
0.065164916792468));
#5703=CARTESIAN_POINT('Ctrl Pts',(0.0412904479475092,0.0987224751365548,
0.0653090151899699));
#5704=CARTESIAN_POINT('Ctrl Pts',(0.0411335425015076,0.0992177720348636,
0.0654121811456859));
#5705=CARTESIAN_POINT('Ctrl Pts',(0.0405168708018142,0.100636070492068,
0.0657455865368071));
#5706=CARTESIAN_POINT('Ctrl Pts',(0.0399051826894431,0.101492776063005,
0.0659940175331532));
#5707=CARTESIAN_POINT('Ctrl Pts',(0.0389827504953742,0.102355632371189,
0.0661099450879691));
#5708=CARTESIAN_POINT('Ctrl Pts',(0.0387729524989471,0.10253278562579,0.066125));
#5709=CARTESIAN_POINT('Ctrl Pts',(0.03855,0.1027,0.066125));
#5710=CARTESIAN_POINT('Origin',(0.05605,0.0842,0.003175));
#5711=CARTESIAN_POINT('',(0.06355,0.0842,0.003175));
#5712=CARTESIAN_POINT('',(0.04855,0.0842,0.003175));
#5713=CARTESIAN_POINT('Origin',(0.04355,0.0842,-0.005825));
#5714=CARTESIAN_POINT('',(0.04355,0.0842,-0.009825));
#5715=CARTESIAN_POINT('',(0.04355,0.0842,-0.001825));
#5716=CARTESIAN_POINT('Origin',(0.05605,0.0842,0.048125));
#5717=CARTESIAN_POINT('',(0.04855,0.0842,0.048125));
#5718=CARTESIAN_POINT('',(0.06355,0.0842,0.048125));
#5719=CARTESIAN_POINT('Origin',(0.04355,0.0842,0.057125));
#5720=CARTESIAN_POINT('',(0.04355,0.0842,0.061125));
#5721=CARTESIAN_POINT('',(0.04355,0.0842,0.053125));
#5722=CARTESIAN_POINT('Origin',(0.06355,0.1092,0.008175));
#5723=CARTESIAN_POINT('Origin',(0.03855,0.0842,-0.009825));
#5724=CARTESIAN_POINT('Origin',(0.04855,0.0842,-0.001825));
#5725=CARTESIAN_POINT('Origin',(0.03855,0.1092,0.061125));
#5726=CARTESIAN_POINT('Origin',(0.04855,0.0842,0.053125));
#5727=CARTESIAN_POINT('Origin',(0.06355,0.0842,0.043125));
#6303=UNCERTAINTY_MEASURE_WITH_UNIT(LENGTH_MEASURE(1.E-5),#6349,
'DISTANCE_ACCURACY_VALUE',
'Maximum model space distance between geometric entities at asserted c
onnectivities');
#6323=UNCERTAINTY_MEASURE_WITH_UNIT(LENGTH_MEASURE(1.E-5),#6349,
'DISTANCE_ACCURACY_VALUE',
'Maximum model space distance between geometric entities at asserted c
onnectivities');
#6328=(
GEOMETRIC_REPRESENTATION_CONTEXT(3)
GLOBAL_UNCERTAINTY_ASSIGNED_CONTEXT((#6303))
GLOBAL_UNIT_ASSIGNED_CONTEXT((#6349,#6350,#6351))
REPRESENTATION_CONTEXT('','3D')
);
#6348=(
GEOMETRIC_REPRESENTATION_CONTEXT(3)
GLOBAL_UNCERTAINTY_ASSIGNED_CONTEXT((#6323))
GLOBAL_UNIT_ASSIGNED_CONTEXT((#6349,#6350,#6351))
REPRESENTATION_CONTEXT('','3D')
);
#6349=(
LENGTH_UNIT()
NAMED_UNIT(*)
SI_UNIT($,.METRE.)
);
#6350=(
NAMED_UNIT(*)
PLANE_ANGLE_UNIT()
SI_UNIT($,.RADIAN.)
);
#6351=(
NAMED_UNIT(*)
SI_UNIT($,.STERADIAN.)
SOLID_ANGLE_UNIT()
);
#6356=SHAPE_DEFINITION_REPRESENTATION(#6380,#6480);
#6380=PRODUCT_DEFINITION_SHAPE('',$,#6505);
#6480=SHAPE_REPRESENTATION('',(#3642),#6328);
#6500=PRODUCT_DEFINITION_CONTEXT('part definition',#6574,'design');
#6505=PRODUCT_DEFINITION('Back Right Z Mount','Back Right Z Mount',#6529,
#6500);
#6529=PRODUCT_DEFINITION_FORMATION('',$,#6580);
#6574=APPLICATION_CONTEXT('Managed model based 3d engineering');
#6575=PRODUCT_CONTEXT('part definition',#6574,'mechanical');
#6580=PRODUCT('Back Right Z Mount','Back Right Z Mount',
'LEGAL AND USAGE DISCLAIMER: this Data/Model is provided \X2\201C\X0\A
S IS\X2\201D\X0\ for informational and representational only. It is a 
geometric approximation and is NOT engineered, certified, or guarantee
d for dimensional accuracy, exact tolerances, or production-level prec
ision. Vendor disclaims all implied warranties including fitness for a
 particular purpose. DO NOT USE FOR DIRECT PHYSICAL MANUFACTURING, AUT
OMATED PRODUCTION, OR SAFETY-CRITICAL SYSTEMS without independent engi
neering verification and resolution of any design discrepancies.',(#6575));
#6601=PRESENTATION_STYLE_ASSIGNMENT((#6607));
#6607=SURFACE_STYLE_USAGE(.BOTH.,#6613);
#6613=SURFACE_SIDE_STYLE('',(#6619));
#6619=SURFACE_STYLE_FILL_AREA(#6625);
#6625=FILL_AREA_STYLE('Opaque(179,179,179)',(#6631));
#6631=FILL_AREA_STYLE_COLOUR('Opaque(179,179,179)',#6637);
#6637=COLOUR_RGB('Opaque(179,179,179)',0.701960784313725,0.701960784313725,
0.701960784313725);
ENDSEC;
END-ISO-10303-21;
